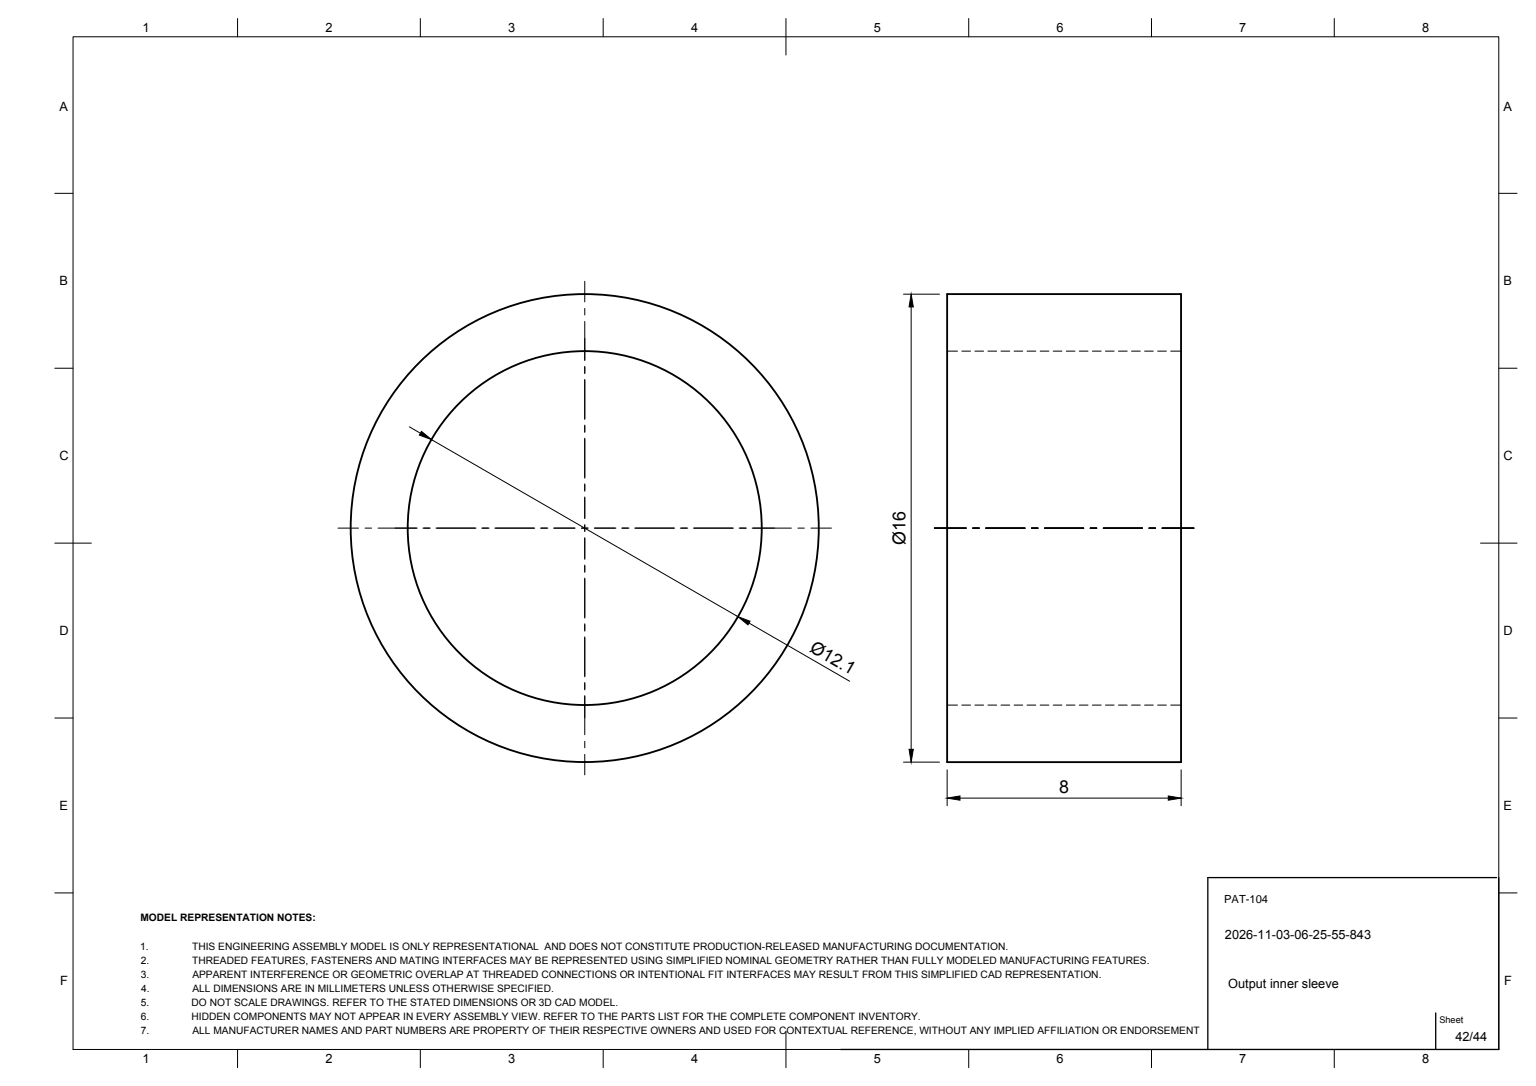
ISO-10303-21;
HEADER;
/* Generated by software containing ST-Developer
 * from STEP Tools, Inc. (www.steptools.com) 
 */

FILE_DESCRIPTION(
/* description */ ('Timing belt drive module 2 mm Pitch Timing 20T-40T'),

/* implementation_level */ '2;1');

FILE_NAME(
/* name */ 'Output inner sleeve.step',
/* time_stamp */ '2026-10-28T03:25:12-07:00',
/* author */ (''),
/* organization */ (''),
/* preprocessor_version */ 'ST-DEVELOPER v20.2',
/* originating_system */ 'Autodesk Translation Framework v15.17.0.0',
/* authorisation */ '');

FILE_SCHEMA (('AUTOMOTIVE_DESIGN { 1 0 10303 214 3 1 1 }'));
ENDSEC;

DATA;
#10=MECHANICAL_DESIGN_GEOMETRIC_PRESENTATION_REPRESENTATION('',(#576),#17830);
#475=SHAPE_REPRESENTATION_RELATIONSHIP('SRR','None',#18049,#518);
#518=ADVANCED_BREP_SHAPE_REPRESENTATION('',(#632),#17824);
#576=STYLED_ITEM('',(#18310),#632);
#632=MANIFOLD_SOLID_BREP('Body1',#9035);
#757=FACE_BOUND('',#2003,.T.);
#758=FACE_BOUND('',#2005,.T.);
#938=PLANE('',#10435);
#939=PLANE('',#10436);
#1359=FACE_OUTER_BOUND('',#2000,.T.);
#1360=FACE_OUTER_BOUND('',#2001,.T.);
#1361=FACE_OUTER_BOUND('',#2002,.T.);
#1362=FACE_OUTER_BOUND('',#2004,.T.);
#2000=EDGE_LOOP('',(#7521,#7522,#7523,#7524));
#2001=EDGE_LOOP('',(#7525,#7526,#7527,#7528));
#2002=EDGE_LOOP('',(#7529));
#2003=EDGE_LOOP('',(#7530));
#2004=EDGE_LOOP('',(#7531));
#2005=EDGE_LOOP('',(#7532));
#2602=CIRCLE('',#10430,0.605);
#2603=CIRCLE('',#10431,0.605);
#2604=CIRCLE('',#10433,0.8);
#2605=CIRCLE('',#10434,0.8);
#3148=LINE('',#16713,#3626);
#3149=LINE('',#16719,#3627);
#3626=VECTOR('',#12997,0.605);
#3627=VECTOR('',#13004,0.8);
#4347=VERTEX_POINT('',#16710);
#4348=VERTEX_POINT('',#16712);
#4349=VERTEX_POINT('',#16716);
#4350=VERTEX_POINT('',#16718);
#5443=EDGE_CURVE('',#4347,#4347,#2602,.T.);
#5444=EDGE_CURVE('',#4347,#4348,#3148,.T.);
#5445=EDGE_CURVE('',#4348,#4348,#2603,.T.);
#5446=EDGE_CURVE('',#4349,#4349,#2604,.T.);
#5447=EDGE_CURVE('',#4349,#4350,#3149,.T.);
#5448=EDGE_CURVE('',#4350,#4350,#2605,.T.);
#7521=ORIENTED_EDGE('',*,*,#5443,.F.);
#7522=ORIENTED_EDGE('',*,*,#5444,.T.);
#7523=ORIENTED_EDGE('',*,*,#5445,.T.);
#7524=ORIENTED_EDGE('',*,*,#5444,.F.);
#7525=ORIENTED_EDGE('',*,*,#5446,.F.);
#7526=ORIENTED_EDGE('',*,*,#5447,.T.);
#7527=ORIENTED_EDGE('',*,*,#5448,.T.);
#7528=ORIENTED_EDGE('',*,*,#5447,.F.);
#7529=ORIENTED_EDGE('',*,*,#5446,.T.);
#7530=ORIENTED_EDGE('',*,*,#5443,.T.);
#7531=ORIENTED_EDGE('',*,*,#5448,.F.);
#7532=ORIENTED_EDGE('',*,*,#5445,.F.);
#8364=CYLINDRICAL_SURFACE('',#10429,0.605);
#8365=CYLINDRICAL_SURFACE('',#10432,0.8);
#8857=ADVANCED_FACE('',(#1359),#8364,.F.);
#8858=ADVANCED_FACE('',(#1360),#8365,.T.);
#8859=ADVANCED_FACE('',(#1361,#757),#938,.T.);
#8860=ADVANCED_FACE('',(#1362,#758),#939,.F.);
#9035=CLOSED_SHELL('',(#8857,#8858,#8859,#8860));
#10428=AXIS2_PLACEMENT_3D('',#16708,#12991,#12992);
#10429=AXIS2_PLACEMENT_3D('',#16709,#12993,#12994);
#10430=AXIS2_PLACEMENT_3D('',#16711,#12995,#12996);
#10431=AXIS2_PLACEMENT_3D('',#16714,#12998,#12999);
#10432=AXIS2_PLACEMENT_3D('',#16715,#13000,#13001);
#10433=AXIS2_PLACEMENT_3D('',#16717,#13002,#13003);
#10434=AXIS2_PLACEMENT_3D('',#16720,#13005,#13006);
#10435=AXIS2_PLACEMENT_3D('',#16721,#13007,#13008);
#10436=AXIS2_PLACEMENT_3D('',#16722,#13009,#13010);
#12991=DIRECTION('axis',(0.,0.,1.));
#12992=DIRECTION('refdir',(1.,0.,0.));
#12993=DIRECTION('center_axis',(0.,1.,0.));
#12994=DIRECTION('ref_axis',(1.,0.,0.));
#12995=DIRECTION('center_axis',(0.,-1.,0.));
#12996=DIRECTION('ref_axis',(1.,0.,0.));
#12997=DIRECTION('',(0.,-1.,0.));
#12998=DIRECTION('center_axis',(0.,-1.,0.));
#12999=DIRECTION('ref_axis',(1.,0.,0.));
#13000=DIRECTION('center_axis',(0.,1.,0.));
#13001=DIRECTION('ref_axis',(1.,0.,0.));
#13002=DIRECTION('center_axis',(0.,1.,0.));
#13003=DIRECTION('ref_axis',(1.,0.,0.));
#13004=DIRECTION('',(0.,-1.,0.));
#13005=DIRECTION('center_axis',(0.,1.,0.));
#13006=DIRECTION('ref_axis',(1.,0.,0.));
#13007=DIRECTION('center_axis',(0.,1.,0.));
#13008=DIRECTION('ref_axis',(1.,0.,0.));
#13009=DIRECTION('center_axis',(0.,1.,0.));
#13010=DIRECTION('ref_axis',(1.,0.,0.));
#16708=CARTESIAN_POINT('',(0.,0.,0.));
#16709=CARTESIAN_POINT('Origin',(6.97091003018116,-0.4,7.));
#16710=CARTESIAN_POINT('',(6.36591003018116,0.4,7.));
#16711=CARTESIAN_POINT('Origin',(6.97091003018116,0.4,7.));
#16712=CARTESIAN_POINT('',(6.36591003018116,-0.4,7.));
#16713=CARTESIAN_POINT('',(6.36591003018116,-0.4,7.));
#16714=CARTESIAN_POINT('Origin',(6.97091003018116,-0.4,7.));
#16715=CARTESIAN_POINT('Origin',(6.97091003018116,-0.4,7.));
#16716=CARTESIAN_POINT('',(6.17091003018116,0.4,7.));
#16717=CARTESIAN_POINT('Origin',(6.97091003018116,0.4,7.));
#16718=CARTESIAN_POINT('',(6.17091003018116,-0.4,7.));
#16719=CARTESIAN_POINT('',(6.17091003018116,-0.4,7.));
#16720=CARTESIAN_POINT('Origin',(6.97091003018116,-0.4,7.));
#16721=CARTESIAN_POINT('Origin',(6.97091003018116,0.4,7.));
#16722=CARTESIAN_POINT('Origin',(6.97091003018116,-0.4,7.));
#17774=UNCERTAINTY_MEASURE_WITH_UNIT(LENGTH_MEASURE(0.001),#17831,
'DISTANCE_ACCURACY_VALUE',
'Maximum model space distance between geometric entities at asserted c
onnectivities');
#17780=UNCERTAINTY_MEASURE_WITH_UNIT(LENGTH_MEASURE(0.001),#17831,
'DISTANCE_ACCURACY_VALUE',
'Maximum model space distance between geometric entities at asserted c
onnectivities');
#17824=(
GEOMETRIC_REPRESENTATION_CONTEXT(3)
GLOBAL_UNCERTAINTY_ASSIGNED_CONTEXT((#17774))
GLOBAL_UNIT_ASSIGNED_CONTEXT((#17831,#17833,#17834))
REPRESENTATION_CONTEXT('','3D')
);
#17830=(
GEOMETRIC_REPRESENTATION_CONTEXT(3)
GLOBAL_UNCERTAINTY_ASSIGNED_CONTEXT((#17780))
GLOBAL_UNIT_ASSIGNED_CONTEXT((#17831,#17833,#17834))
REPRESENTATION_CONTEXT('','3D')
);
#17831=(
LENGTH_UNIT()
NAMED_UNIT(*)
SI_UNIT(.CENTI.,.METRE.)
);
#17833=(
NAMED_UNIT(*)
PLANE_ANGLE_UNIT()
SI_UNIT($,.RADIAN.)
);
#17834=(
NAMED_UNIT(*)
SI_UNIT($,.STERADIAN.)
SOLID_ANGLE_UNIT()
);
#17878=SHAPE_DEFINITION_REPRESENTATION(#17937,#18049);
#17937=PRODUCT_DEFINITION_SHAPE('',$,#18099);
#18049=SHAPE_REPRESENTATION('',(#10428),#17824);
#18055=PRODUCT_DEFINITION_CONTEXT('part definition',#18204,'design');
#18099=PRODUCT_DEFINITION('Output inner sleeve','Output inner sleeve',#18148,
#18055);
#18148=PRODUCT_DEFINITION_FORMATION('',$,#18249);
#18204=APPLICATION_CONTEXT(
'Core Data for Automotive Mechanical Design Process');
#18205=PRODUCT_CONTEXT('part definition',#18204,'mechanical');
#18249=PRODUCT('Output inner sleeve','Output inner sleeve',
'Output inner sleeve',(#18205));
#18304=COLOUR_RGB('Sky Blue',0.24,0.69,0.87);
#18305=FILL_AREA_STYLE_COLOUR('',#18304);
#18306=FILL_AREA_STYLE('',(#18305));
#18307=SURFACE_STYLE_FILL_AREA(#18306);
#18308=SURFACE_SIDE_STYLE('',(#18307));
#18309=SURFACE_STYLE_USAGE(.BOTH.,#18308);
#18310=PRESENTATION_STYLE_ASSIGNMENT((#18309));
ENDSEC;
END-ISO-10303-21;
